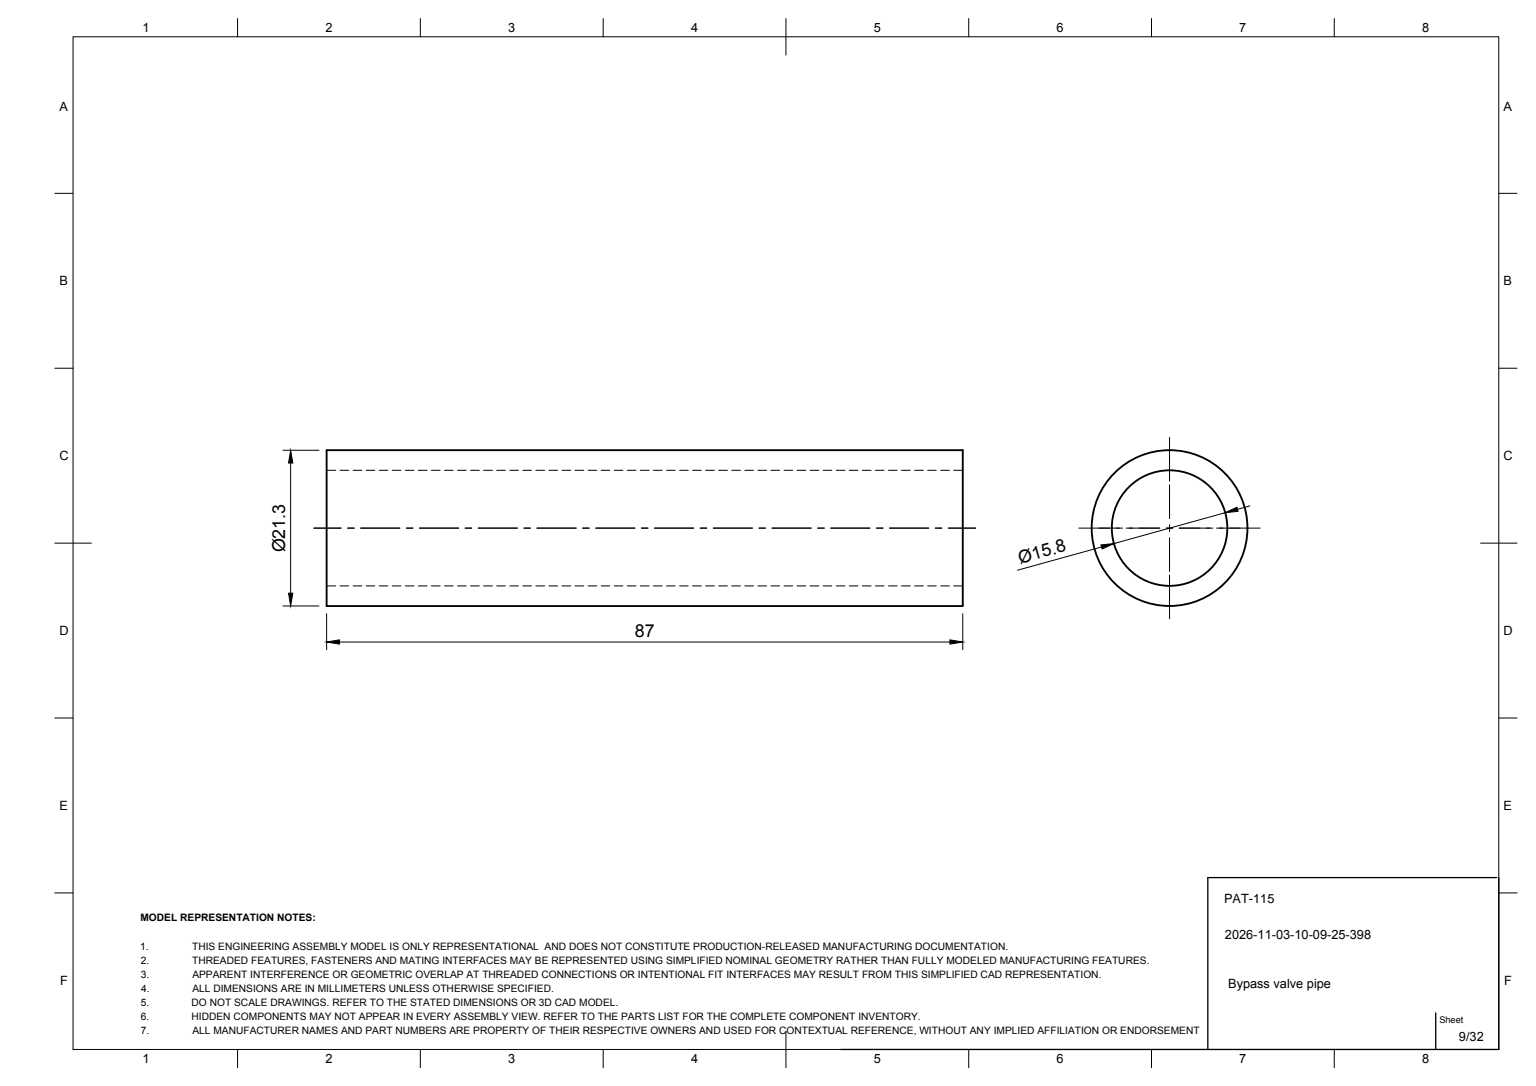
ISO-10303-21;
HEADER;
/* Generated by software containing ST-Developer
 * from STEP Tools, Inc. (www.steptools.com) 
 */

FILE_DESCRIPTION(
/* description */ ('Union bypass pipe loop'),
/* implementation_level */ '2;1');

FILE_NAME(
/* name */ 'Bypass valve pipe.step',
/* time_stamp */ '2026-10-27T21:00:29-07:00',
/* author */ (''),
/* organization */ (''),
/* preprocessor_version */ 'ST-DEVELOPER v20.2',
/* originating_system */ 'Autodesk Translation Framework v15.17.0.0',
/* authorisation */ '');

FILE_SCHEMA (('AUTOMOTIVE_DESIGN { 1 0 10303 214 3 1 1 }'));
ENDSEC;

DATA;
#10=MECHANICAL_DESIGN_GEOMETRIC_PRESENTATION_REPRESENTATION('',(#463),#10095);
#399=SHAPE_REPRESENTATION_RELATIONSHIP('SRR','None',#10268,#431);
#431=ADVANCED_BREP_SHAPE_REPRESENTATION('',(#493),#10080);
#463=STYLED_ITEM('',(#10486),#493);
#493=MANIFOLD_SOLID_BREP('Body1',#5536);
#586=FACE_BOUND('',#1425,.T.);
#587=FACE_BOUND('',#1427,.T.);
#736=PLANE('',#6309);
#737=PLANE('',#6310);
#1015=FACE_OUTER_BOUND('',#1422,.T.);
#1016=FACE_OUTER_BOUND('',#1423,.T.);
#1017=FACE_OUTER_BOUND('',#1424,.T.);
#1018=FACE_OUTER_BOUND('',#1426,.T.);
#1422=EDGE_LOOP('',(#4464,#4465,#4466,#4467));
#1423=EDGE_LOOP('',(#4468,#4469,#4470,#4471));
#1424=EDGE_LOOP('',(#4472));
#1425=EDGE_LOOP('',(#4473));
#1426=EDGE_LOOP('',(#4474));
#1427=EDGE_LOOP('',(#4475));
#1813=LINE('',#9287,#2189);
#1814=LINE('',#9293,#2190);
#2189=VECTOR('',#7609,0.79);
#2190=VECTOR('',#7616,1.065);
#2522=CIRCLE('',#6304,0.79);
#2523=CIRCLE('',#6305,0.79);
#2524=CIRCLE('',#6307,1.065);
#2525=CIRCLE('',#6308,1.065);
#2866=VERTEX_POINT('',#9284);
#2867=VERTEX_POINT('',#9286);
#2868=VERTEX_POINT('',#9290);
#2869=VERTEX_POINT('',#9292);
#3430=EDGE_CURVE('',#2866,#2866,#2522,.T.);
#3431=EDGE_CURVE('',#2866,#2867,#1813,.T.);
#3432=EDGE_CURVE('',#2867,#2867,#2523,.T.);
#3433=EDGE_CURVE('',#2868,#2868,#2524,.T.);
#3434=EDGE_CURVE('',#2868,#2869,#1814,.T.);
#3435=EDGE_CURVE('',#2869,#2869,#2525,.T.);
#4464=ORIENTED_EDGE('',*,*,#3430,.F.);
#4465=ORIENTED_EDGE('',*,*,#3431,.T.);
#4466=ORIENTED_EDGE('',*,*,#3432,.T.);
#4467=ORIENTED_EDGE('',*,*,#3431,.F.);
#4468=ORIENTED_EDGE('',*,*,#3433,.F.);
#4469=ORIENTED_EDGE('',*,*,#3434,.T.);
#4470=ORIENTED_EDGE('',*,*,#3435,.T.);
#4471=ORIENTED_EDGE('',*,*,#3434,.F.);
#4472=ORIENTED_EDGE('',*,*,#3433,.T.);
#4473=ORIENTED_EDGE('',*,*,#3430,.T.);
#4474=ORIENTED_EDGE('',*,*,#3435,.F.);
#4475=ORIENTED_EDGE('',*,*,#3432,.F.);
#5145=CYLINDRICAL_SURFACE('',#6303,0.79);
#5146=CYLINDRICAL_SURFACE('',#6306,1.065);
#5364=ADVANCED_FACE('',(#1015),#5145,.F.);
#5365=ADVANCED_FACE('',(#1016),#5146,.T.);
#5366=ADVANCED_FACE('',(#1017,#586),#736,.T.);
#5367=ADVANCED_FACE('',(#1018,#587),#737,.F.);
#5536=CLOSED_SHELL('',(#5364,#5365,#5366,#5367));
#6302=AXIS2_PLACEMENT_3D('',#9282,#7603,#7604);
#6303=AXIS2_PLACEMENT_3D('',#9283,#7605,#7606);
#6304=AXIS2_PLACEMENT_3D('',#9285,#7607,#7608);
#6305=AXIS2_PLACEMENT_3D('',#9288,#7610,#7611);
#6306=AXIS2_PLACEMENT_3D('',#9289,#7612,#7613);
#6307=AXIS2_PLACEMENT_3D('',#9291,#7614,#7615);
#6308=AXIS2_PLACEMENT_3D('',#9294,#7617,#7618);
#6309=AXIS2_PLACEMENT_3D('',#9295,#7619,#7620);
#6310=AXIS2_PLACEMENT_3D('',#9296,#7621,#7622);
#7603=DIRECTION('axis',(0.,0.,1.));
#7604=DIRECTION('refdir',(1.,0.,0.));
#7605=DIRECTION('center_axis',(1.,0.,0.));
#7606=DIRECTION('ref_axis',(0.,0.,-1.));
#7607=DIRECTION('center_axis',(-1.,0.,0.));
#7608=DIRECTION('ref_axis',(0.,0.,-1.));
#7609=DIRECTION('',(-1.,0.,0.));
#7610=DIRECTION('center_axis',(-1.,0.,0.));
#7611=DIRECTION('ref_axis',(0.,0.,-1.));
#7612=DIRECTION('center_axis',(1.,0.,0.));
#7613=DIRECTION('ref_axis',(0.,0.,-1.));
#7614=DIRECTION('center_axis',(1.,0.,0.));
#7615=DIRECTION('ref_axis',(0.,0.,-1.));
#7616=DIRECTION('',(-1.,0.,0.));
#7617=DIRECTION('center_axis',(1.,0.,0.));
#7618=DIRECTION('ref_axis',(0.,0.,-1.));
#7619=DIRECTION('center_axis',(1.,0.,0.));
#7620=DIRECTION('ref_axis',(0.,0.,-1.));
#7621=DIRECTION('center_axis',(1.,0.,0.));
#7622=DIRECTION('ref_axis',(0.,0.,-1.));
#9282=CARTESIAN_POINT('',(0.,0.,0.));
#9283=CARTESIAN_POINT('Origin',(-10.5,-12.,5.));
#9284=CARTESIAN_POINT('',(-1.8,-12.,5.79));
#9285=CARTESIAN_POINT('Origin',(-1.8,-12.,5.));
#9286=CARTESIAN_POINT('',(-10.5,-12.,5.79));
#9287=CARTESIAN_POINT('',(-10.5,-12.,5.79));
#9288=CARTESIAN_POINT('Origin',(-10.5,-12.,5.));
#9289=CARTESIAN_POINT('Origin',(-10.5,-12.,5.));
#9290=CARTESIAN_POINT('',(-1.8,-12.,6.065));
#9291=CARTESIAN_POINT('Origin',(-1.8,-12.,5.));
#9292=CARTESIAN_POINT('',(-10.5,-12.,6.065));
#9293=CARTESIAN_POINT('',(-10.5,-12.,6.065));
#9294=CARTESIAN_POINT('Origin',(-10.5,-12.,5.));
#9295=CARTESIAN_POINT('Origin',(-1.8,-12.,5.));
#9296=CARTESIAN_POINT('Origin',(-10.5,-12.,5.));
#10043=UNCERTAINTY_MEASURE_WITH_UNIT(LENGTH_MEASURE(0.001),#10096,
'DISTANCE_ACCURACY_VALUE',
'Maximum model space distance between geometric entities at asserted c
onnectivities');
#10058=UNCERTAINTY_MEASURE_WITH_UNIT(LENGTH_MEASURE(0.001),#10096,
'DISTANCE_ACCURACY_VALUE',
'Maximum model space distance between geometric entities at asserted c
onnectivities');
#10080=(
GEOMETRIC_REPRESENTATION_CONTEXT(3)
GLOBAL_UNCERTAINTY_ASSIGNED_CONTEXT((#10043))
GLOBAL_UNIT_ASSIGNED_CONTEXT((#10096,#10098,#10099))
REPRESENTATION_CONTEXT('','3D')
);
#10095=(
GEOMETRIC_REPRESENTATION_CONTEXT(3)
GLOBAL_UNCERTAINTY_ASSIGNED_CONTEXT((#10058))
GLOBAL_UNIT_ASSIGNED_CONTEXT((#10096,#10098,#10099))
REPRESENTATION_CONTEXT('','3D')
);
#10096=(
LENGTH_UNIT()
NAMED_UNIT(*)
SI_UNIT(.CENTI.,.METRE.)
);
#10098=(
NAMED_UNIT(*)
PLANE_ANGLE_UNIT()
SI_UNIT($,.RADIAN.)
);
#10099=(
NAMED_UNIT(*)
SI_UNIT($,.STERADIAN.)
SOLID_ANGLE_UNIT()
);
#10121=SHAPE_DEFINITION_REPRESENTATION(#10192,#10268);
#10192=PRODUCT_DEFINITION_SHAPE('',$,#10305);
#10268=SHAPE_REPRESENTATION('',(#6302),#10080);
#10283=PRODUCT_DEFINITION_CONTEXT('part definition',#10393,'design');
#10305=PRODUCT_DEFINITION('Bypass valve pipe','Bypass valve pipe',#10341,
#10283);
#10341=PRODUCT_DEFINITION_FORMATION('',$,#10416);
#10393=APPLICATION_CONTEXT(
'Core Data for Automotive Mechanical Design Process');
#10394=PRODUCT_CONTEXT('part definition',#10393,'mechanical');
#10416=PRODUCT('Bypass valve pipe','Bypass valve pipe',
'Bypass valve pipe',(#10394));
#10480=COLOUR_RGB('Light Blue',0.38,0.62,0.78);
#10481=FILL_AREA_STYLE_COLOUR('',#10480);
#10482=FILL_AREA_STYLE('',(#10481));
#10483=SURFACE_STYLE_FILL_AREA(#10482);
#10484=SURFACE_SIDE_STYLE('',(#10483));
#10485=SURFACE_STYLE_USAGE(.BOTH.,#10484);
#10486=PRESENTATION_STYLE_ASSIGNMENT((#10485));
ENDSEC;
END-ISO-10303-21;
